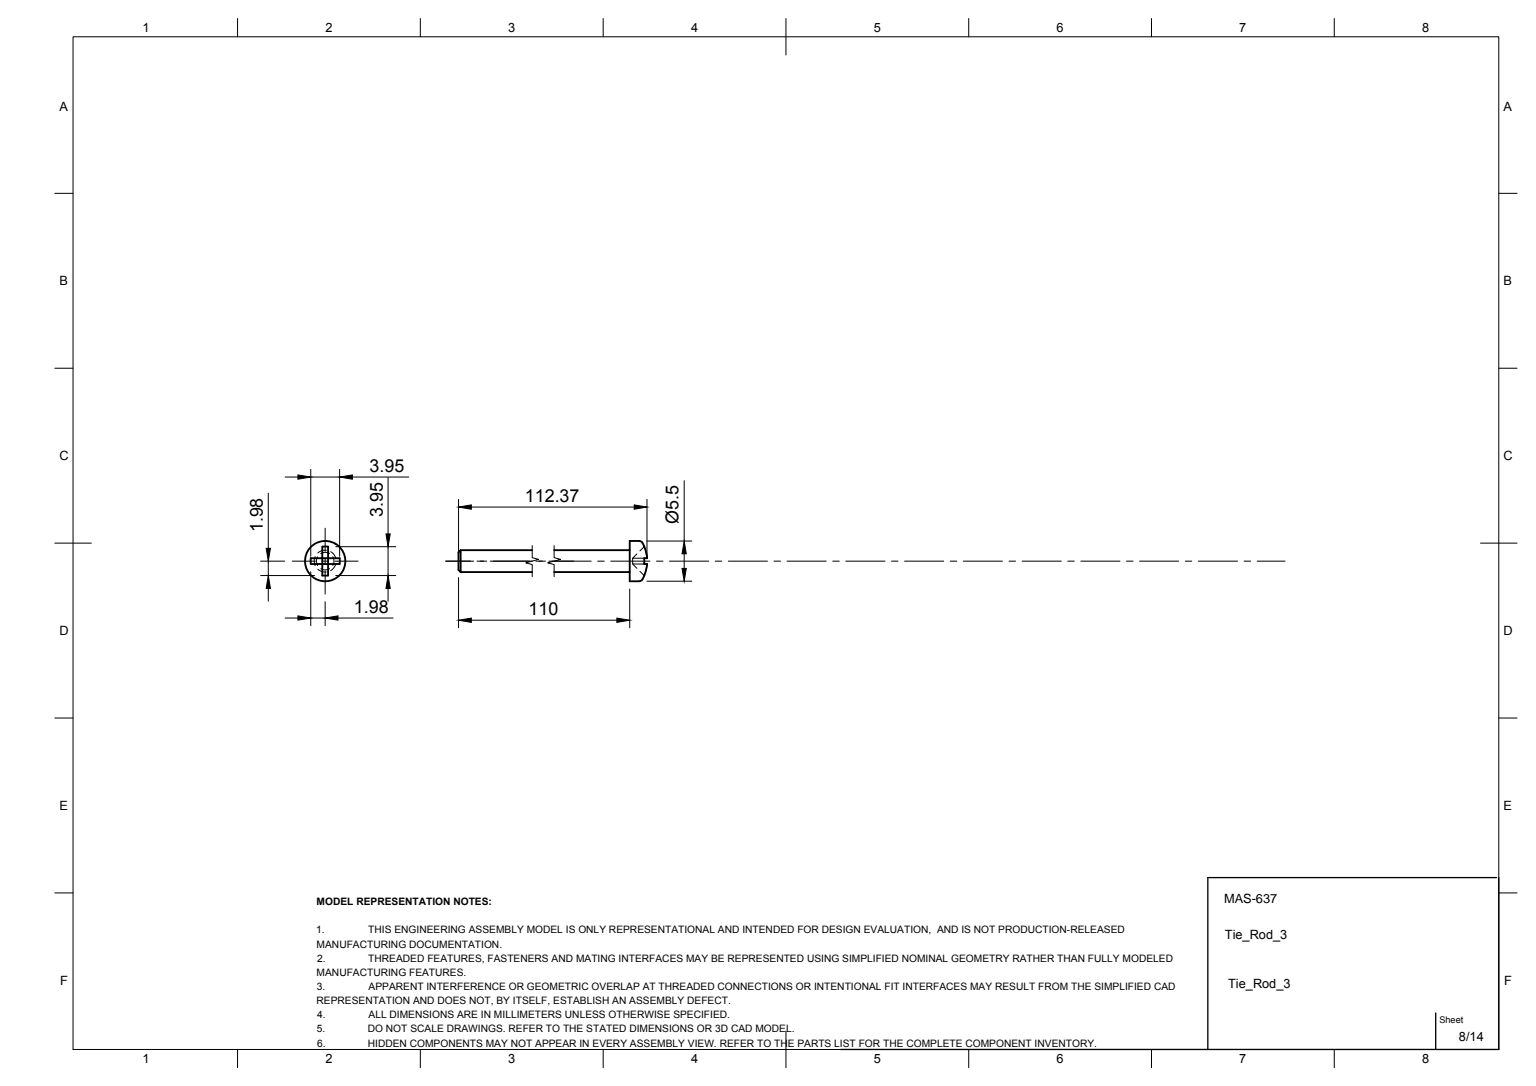
ISO-10303-21;
HEADER;
FILE_DESCRIPTION((''),'2;1');
FILE_NAME('Tie_Rod_3.step','2026-10-09T10:11:57-07:00',(''),(''),'','','');
FILE_SCHEMA (('AUTOMOTIVE_DESIGN { 1 0 10303 214 3 1 1 }'));
ENDSEC;
DATA;
#10=MECHANICAL_DESIGN_GEOMETRIC_PRESENTATION_REPRESENTATION('',(#128),#13510);
#73=SPHERICAL_SURFACE('',#8150,5.) ;
#98=SHAPE_REPRESENTATION_RELATIONSHIP('SRR','None',#13568,#113) ;
#113=ADVANCED_BREP_SHAPE_REPRESENTATION('',(#160),#13500) ;
#128=STYLED_ITEM('',(#13650),#160) ;
#160=MANIFOLD_SOLID_BREP('Body1',#7377) ;
#242=FACE_BOUND('',#1414,.T.) ;
#382=PLANE('',#8135) ;
#383=PLANE('',#8136) ;
#384=PLANE('',#8137) ;
#385=PLANE('',#8139) ;
#386=PLANE('',#8141) ;
#387=PLANE('',#8144) ;
#388=PLANE('',#8146) ;
#389=PLANE('',#8148) ;
#390=PLANE('',#8158) ;
#391=PLANE('',#8159) ;
#392=PLANE('',#8160) ;
#393=PLANE('',#8161) ;
#394=PLANE('',#8162) ;
#395=PLANE('',#8163) ;
#396=PLANE('',#8164) ;
#500=TOROIDAL_SURFACE('',#8124,2.25,0.5) ;
#636=CYLINDRICAL_SURFACE('',#8128,2.75) ;
#637=CYLINDRICAL_SURFACE('',#8130,1.5) ;
#906=FACE_OUTER_BOUND('',#1409,.T.) ;
#907=FACE_OUTER_BOUND('',#1410,.T.) ;
#908=FACE_OUTER_BOUND('',#1411,.T.) ;
#909=FACE_OUTER_BOUND('',#1412,.T.) ;
#910=FACE_OUTER_BOUND('',#1413,.T.) ;
#911=FACE_OUTER_BOUND('',#1415,.T.) ;
#912=FACE_OUTER_BOUND('',#1416,.T.) ;
#913=FACE_OUTER_BOUND('',#1417,.T.) ;
#914=FACE_OUTER_BOUND('',#1418,.T.) ;
#915=FACE_OUTER_BOUND('',#1419,.T.) ;
#916=FACE_OUTER_BOUND('',#1420,.T.) ;
#917=FACE_OUTER_BOUND('',#1421,.T.) ;
#918=FACE_OUTER_BOUND('',#1422,.T.) ;
#919=FACE_OUTER_BOUND('',#1423,.T.) ;
#920=FACE_OUTER_BOUND('',#1424,.T.) ;
#921=FACE_OUTER_BOUND('',#1425,.T.) ;
#922=FACE_OUTER_BOUND('',#1426,.T.) ;
#923=FACE_OUTER_BOUND('',#1427,.T.) ;
#924=FACE_OUTER_BOUND('',#1428,.T.) ;
#925=FACE_OUTER_BOUND('',#1429,.T.) ;
#1409=EDGE_LOOP('',(#6066,#6067,#6068,#6069)) ;
#1410=EDGE_LOOP('',(#6070,#6071,#6072,#6073)) ;
#1411=EDGE_LOOP('',(#6074,#6075,#6076,#6077)) ;
#1412=EDGE_LOOP('',(#6078,#6079,#6080,#6081)) ;
#1413=EDGE_LOOP('',(#6082)) ;
#1414=EDGE_LOOP('',(#6083)) ;
#1415=EDGE_LOOP('',(#6084)) ;
#1416=EDGE_LOOP('',(#6085,#6086,#6087,#6088)) ;
#1417=EDGE_LOOP('',(#6089,#6090,#6091,#6092)) ;
#1418=EDGE_LOOP('',(#6093,#6094,#6095,#6096)) ;
#1419=EDGE_LOOP('',(#6097,#6098,#6099)) ;
#1420=EDGE_LOOP('',(#6100,#6101,#6102)) ;
#1421=EDGE_LOOP('',(#6103,#6104,#6105)) ;
#1422=EDGE_LOOP('',(#6106,#6107,#6108,#6109,#6110,#6111,#6112,#6113,#6114,
#6115,#6116,#6117,#6118,#6119,#6120,#6121)) ;
#1423=EDGE_LOOP('',(#6122,#6123,#6124)) ;
#1424=EDGE_LOOP('',(#6125,#6126,#6127,#6128)) ;
#1425=EDGE_LOOP('',(#6129,#6130,#6131)) ;
#1426=EDGE_LOOP('',(#6132,#6133,#6134)) ;
#1427=EDGE_LOOP('',(#6135,#6136,#6137,#6138)) ;
#1428=EDGE_LOOP('',(#6139,#6140,#6141)) ;
#1429=EDGE_LOOP('',(#6142,#6143,#6144,#6145)) ;
#1944=LINE('',#12588,#2438) ;
#1945=LINE('',#12593,#2439) ;
#1946=LINE('',#12597,#2440) ;
#1947=LINE('',#12604,#2441) ;
#1948=LINE('',#12606,#2442) ;
#1949=LINE('',#12608,#2443) ;
#1950=LINE('',#12615,#2444) ;
#1951=LINE('',#12617,#2445) ;
#1952=LINE('',#12618,#2446) ;
#1953=LINE('',#12621,#2447) ;
#1954=LINE('',#12627,#2448) ;
#1955=LINE('',#12632,#2449) ;
#1956=LINE('',#12636,#2450) ;
#1957=LINE('',#12650,#2451) ;
#1958=LINE('',#12652,#2452) ;
#1959=LINE('',#12653,#2453) ;
#1960=LINE('',#12656,#2454) ;
#1961=LINE('',#12658,#2455) ;
#1962=LINE('',#12659,#2456) ;
#2438=VECTOR('',#9982,2.75) ;
#2439=VECTOR('',#9987,1.5) ;
#2440=VECTOR('',#9992,1.2) ;
#2441=VECTOR('',#10001,1.00000000000035) ;
#2442=VECTOR('',#10002,0.99999999999962) ;
#2443=VECTOR('',#10003,1.00000000000035) ;
#2444=VECTOR('',#10010,1.00000000000035) ;
#2445=VECTOR('',#10011,0.99999999999962) ;
#2446=VECTOR('',#10012,1.00000000000035) ;
#2447=VECTOR('',#10015,1.) ;
#2448=VECTOR('',#10022,1.) ;
#2449=VECTOR('',#10029,1.) ;
#2450=VECTOR('',#10034,1.) ;
#2451=VECTOR('',#10053,1.00000000000035) ;
#2452=VECTOR('',#10056,1.00000000000035) ;
#2453=VECTOR('',#10057,0.99999999999962) ;
#2454=VECTOR('',#10062,1.00000000000035) ;
#2455=VECTOR('',#10065,0.99999999999962) ;
#2456=VECTOR('',#10066,1.00000000000035) ;
#2940=CIRCLE('',#8125,2.75) ;
#2941=CIRCLE('',#8126,0.5) ;
#2942=CIRCLE('',#8127,2.5) ;
#2943=CIRCLE('',#8129,2.75) ;
#2944=CIRCLE('',#8131,1.5) ;
#2945=CIRCLE('',#8132,1.5) ;
#2946=CIRCLE('',#8134,1.2) ;
#2947=CIRCLE('',#8138,4.64997589841126) ;
#2948=CIRCLE('',#8140,4.64997589841224) ;
#2949=CIRCLE('',#8142,4.98397431775083) ;
#2950=CIRCLE('',#8143,4.98397431775083) ;
#2951=CIRCLE('',#8145,4.98396179855413) ;
#2952=CIRCLE('',#8147,4.98396179762506) ;
#2953=CIRCLE('',#8149,4.98397431775083) ;
#2954=CIRCLE('',#8151,5.) ;
#2955=CIRCLE('',#8152,4.9839743177518) ;
#2956=CIRCLE('',#8153,4.64973117502146) ;
#2957=CIRCLE('',#8154,4.98397431775041) ;
#2958=CIRCLE('',#8155,4.98397431775041) ;
#2959=CIRCLE('',#8156,4.64973117502146) ;
#2960=CIRCLE('',#8157,4.9839743177518) ;
#3542=VERTEX_POINT('',#12580) ;
#3543=VERTEX_POINT('',#12582) ;
#3544=VERTEX_POINT('',#12586) ;
#3545=VERTEX_POINT('',#12590) ;
#3546=VERTEX_POINT('',#12592) ;
#3547=VERTEX_POINT('',#12596) ;
#3548=VERTEX_POINT('',#12602) ;
#3549=VERTEX_POINT('',#12603) ;
#3550=VERTEX_POINT('',#12605) ;
#3551=VERTEX_POINT('',#12607) ;
#3552=VERTEX_POINT('',#12611) ;
#3553=VERTEX_POINT('',#12612) ;
#3554=VERTEX_POINT('',#12614) ;
#3555=VERTEX_POINT('',#12616) ;
#3556=VERTEX_POINT('',#12620) ;
#3557=VERTEX_POINT('',#12622) ;
#3558=VERTEX_POINT('',#12626) ;
#3559=VERTEX_POINT('',#12630) ;
#3560=VERTEX_POINT('',#12634) ;
#3561=VERTEX_POINT('',#12639) ;
#3562=VERTEX_POINT('',#12641) ;
#3563=VERTEX_POINT('',#12644) ;
#3564=VERTEX_POINT('',#12646) ;
#4420=EDGE_CURVE('',#3542,#3542,#2940,.T.) ;
#4421=EDGE_CURVE('',#3542,#3543,#2941,.T.) ;
#4422=EDGE_CURVE('',#3543,#3543,#2942,.T.) ;
#4423=EDGE_CURVE('',#3544,#3544,#2943,.T.) ;
#4424=EDGE_CURVE('',#3544,#3542,#1944,.T.) ;
#4425=EDGE_CURVE('',#3545,#3545,#2944,.T.) ;
#4426=EDGE_CURVE('',#3545,#3546,#1945,.T.) ;
#4427=EDGE_CURVE('',#3546,#3546,#2945,.T.) ;
#4428=EDGE_CURVE('',#3545,#3547,#1946,.T.) ;
#4429=EDGE_CURVE('',#3547,#3547,#2946,.F.) ;
#4430=EDGE_CURVE('',#3548,#3549,#1947,.T.) ;
#4431=EDGE_CURVE('',#3548,#3550,#1948,.F.) ;
#4432=EDGE_CURVE('',#3550,#3551,#1949,.T.) ;
#4433=EDGE_CURVE('',#3551,#3549,#2947,.T.) ;
#4434=EDGE_CURVE('',#3552,#3553,#2948,.T.) ;
#4435=EDGE_CURVE('',#3552,#3554,#1950,.F.) ;
#4436=EDGE_CURVE('',#3555,#3554,#1951,.F.) ;
#4437=EDGE_CURVE('',#3553,#3555,#1952,.F.) ;
#4438=EDGE_CURVE('',#3550,#3556,#1953,.T.) ;
#4439=EDGE_CURVE('',#3557,#3556,#2949,.F.) ;
#4440=EDGE_CURVE('',#3551,#3557,#2950,.F.) ;
#4441=EDGE_CURVE('',#3554,#3558,#1954,.T.) ;
#4442=EDGE_CURVE('',#3558,#3552,#2951,.T.) ;
#4443=EDGE_CURVE('',#3559,#3549,#2952,.T.) ;
#4444=EDGE_CURVE('',#3548,#3559,#1955,.T.) ;
#4445=EDGE_CURVE('',#3553,#3560,#2953,.F.) ;
#4446=EDGE_CURVE('',#3555,#3560,#1956,.T.) ;
#4447=EDGE_CURVE('',#3543,#3557,#2954,.T.) ;
#4448=EDGE_CURVE('',#3561,#3556,#2955,.T.) ;
#4449=EDGE_CURVE('',#3562,#3561,#2956,.T.) ;
#4450=EDGE_CURVE('',#3562,#3558,#2957,.T.) ;
#4451=EDGE_CURVE('',#3563,#3560,#2958,.T.) ;
#4452=EDGE_CURVE('',#3563,#3564,#2959,.T.) ;
#4453=EDGE_CURVE('',#3564,#3559,#2960,.T.) ;
#4454=EDGE_CURVE('',#3564,#3548,#1957,.F.) ;
#4455=EDGE_CURVE('',#3563,#3555,#1958,.F.) ;
#4456=EDGE_CURVE('',#3555,#3548,#1959,.T.) ;
#4457=EDGE_CURVE('',#3550,#3561,#1960,.T.) ;
#4458=EDGE_CURVE('',#3554,#3550,#1961,.T.) ;
#4459=EDGE_CURVE('',#3554,#3562,#1962,.T.) ;
#6066=ORIENTED_EDGE('',*,*,#4420,.F.) ;
#6067=ORIENTED_EDGE('',*,*,#4421,.T.) ;
#6068=ORIENTED_EDGE('',*,*,#4422,.T.) ;
#6069=ORIENTED_EDGE('',*,*,#4421,.F.) ;
#6070=ORIENTED_EDGE('',*,*,#4423,.F.) ;
#6071=ORIENTED_EDGE('',*,*,#4424,.T.) ;
#6072=ORIENTED_EDGE('',*,*,#4420,.T.) ;
#6073=ORIENTED_EDGE('',*,*,#4424,.F.) ;
#6074=ORIENTED_EDGE('',*,*,#4425,.F.) ;
#6075=ORIENTED_EDGE('',*,*,#4426,.T.) ;
#6076=ORIENTED_EDGE('',*,*,#4427,.T.) ;
#6077=ORIENTED_EDGE('',*,*,#4426,.F.) ;
#6078=ORIENTED_EDGE('',*,*,#4425,.T.) ;
#6079=ORIENTED_EDGE('',*,*,#4428,.T.) ;
#6080=ORIENTED_EDGE('',*,*,#4429,.F.) ;
#6081=ORIENTED_EDGE('',*,*,#4428,.F.) ;
#6082=ORIENTED_EDGE('',*,*,#4423,.T.) ;
#6083=ORIENTED_EDGE('',*,*,#4427,.F.) ;
#6084=ORIENTED_EDGE('',*,*,#4429,.T.) ;
#6085=ORIENTED_EDGE('',*,*,#4430,.F.) ;
#6086=ORIENTED_EDGE('',*,*,#4431,.T.) ;
#6087=ORIENTED_EDGE('',*,*,#4432,.T.) ;
#6088=ORIENTED_EDGE('',*,*,#4433,.T.) ;
#6089=ORIENTED_EDGE('',*,*,#4434,.F.) ;
#6090=ORIENTED_EDGE('',*,*,#4435,.T.) ;
#6091=ORIENTED_EDGE('',*,*,#4436,.F.) ;
#6092=ORIENTED_EDGE('',*,*,#4437,.F.) ;
#6093=ORIENTED_EDGE('',*,*,#4438,.T.) ;
#6094=ORIENTED_EDGE('',*,*,#4439,.F.) ;
#6095=ORIENTED_EDGE('',*,*,#4440,.F.) ;
#6096=ORIENTED_EDGE('',*,*,#4432,.F.) ;
#6097=ORIENTED_EDGE('',*,*,#4441,.F.) ;
#6098=ORIENTED_EDGE('',*,*,#4435,.F.) ;
#6099=ORIENTED_EDGE('',*,*,#4442,.F.) ;
#6100=ORIENTED_EDGE('',*,*,#4430,.T.) ;
#6101=ORIENTED_EDGE('',*,*,#4443,.F.) ;
#6102=ORIENTED_EDGE('',*,*,#4444,.F.) ;
#6103=ORIENTED_EDGE('',*,*,#4445,.F.) ;
#6104=ORIENTED_EDGE('',*,*,#4437,.T.) ;
#6105=ORIENTED_EDGE('',*,*,#4446,.T.) ;
#6106=ORIENTED_EDGE('',*,*,#4422,.F.) ;
#6107=ORIENTED_EDGE('',*,*,#4447,.T.) ;
#6108=ORIENTED_EDGE('',*,*,#4439,.T.) ;
#6109=ORIENTED_EDGE('',*,*,#4448,.F.) ;
#6110=ORIENTED_EDGE('',*,*,#4449,.F.) ;
#6111=ORIENTED_EDGE('',*,*,#4450,.T.) ;
#6112=ORIENTED_EDGE('',*,*,#4442,.T.) ;
#6113=ORIENTED_EDGE('',*,*,#4434,.T.) ;
#6114=ORIENTED_EDGE('',*,*,#4445,.T.) ;
#6115=ORIENTED_EDGE('',*,*,#4451,.F.) ;
#6116=ORIENTED_EDGE('',*,*,#4452,.T.) ;
#6117=ORIENTED_EDGE('',*,*,#4453,.T.) ;
#6118=ORIENTED_EDGE('',*,*,#4443,.T.) ;
#6119=ORIENTED_EDGE('',*,*,#4433,.F.) ;
#6120=ORIENTED_EDGE('',*,*,#4440,.T.) ;
#6121=ORIENTED_EDGE('',*,*,#4447,.F.) ;
#6122=ORIENTED_EDGE('',*,*,#4454,.T.) ;
#6123=ORIENTED_EDGE('',*,*,#4444,.T.) ;
#6124=ORIENTED_EDGE('',*,*,#4453,.F.) ;
#6125=ORIENTED_EDGE('',*,*,#4454,.F.) ;
#6126=ORIENTED_EDGE('',*,*,#4452,.F.) ;
#6127=ORIENTED_EDGE('',*,*,#4455,.T.) ;
#6128=ORIENTED_EDGE('',*,*,#4456,.T.) ;
#6129=ORIENTED_EDGE('',*,*,#4451,.T.) ;
#6130=ORIENTED_EDGE('',*,*,#4446,.F.) ;
#6131=ORIENTED_EDGE('',*,*,#4455,.F.) ;
#6132=ORIENTED_EDGE('',*,*,#4457,.T.) ;
#6133=ORIENTED_EDGE('',*,*,#4448,.T.) ;
#6134=ORIENTED_EDGE('',*,*,#4438,.F.) ;
#6135=ORIENTED_EDGE('',*,*,#4457,.F.) ;
#6136=ORIENTED_EDGE('',*,*,#4458,.F.) ;
#6137=ORIENTED_EDGE('',*,*,#4459,.T.) ;
#6138=ORIENTED_EDGE('',*,*,#4449,.T.) ;
#6139=ORIENTED_EDGE('',*,*,#4441,.T.) ;
#6140=ORIENTED_EDGE('',*,*,#4450,.F.) ;
#6141=ORIENTED_EDGE('',*,*,#4459,.F.) ;
#6142=ORIENTED_EDGE('',*,*,#4458,.T.) ;
#6143=ORIENTED_EDGE('',*,*,#4431,.F.) ;
#6144=ORIENTED_EDGE('',*,*,#4456,.F.) ;
#6145=ORIENTED_EDGE('',*,*,#4436,.T.) ;
#6887=CONICAL_SURFACE('',#8133,1.2,0.785398163397) ;
#7156=ADVANCED_FACE('',(#906),#500,.T.) ;
#7157=ADVANCED_FACE('',(#907),#636,.T.) ;
#7158=ADVANCED_FACE('',(#908),#637,.T.) ;
#7159=ADVANCED_FACE('',(#909),#6887,.T.) ;
#7160=ADVANCED_FACE('',(#910,#242),#382,.T.) ;
#7161=ADVANCED_FACE('',(#911),#383,.T.) ;
#7162=ADVANCED_FACE('',(#912),#384,.T.) ;
#7163=ADVANCED_FACE('',(#913),#385,.F.) ;
#7164=ADVANCED_FACE('',(#914),#386,.F.) ;
#7165=ADVANCED_FACE('',(#915),#387,.F.) ;
#7166=ADVANCED_FACE('',(#916),#388,.T.) ;
#7167=ADVANCED_FACE('',(#917),#389,.T.) ;
#7168=ADVANCED_FACE('',(#918),#73,.T.) ;
#7169=ADVANCED_FACE('',(#919),#390,.T.) ;
#7170=ADVANCED_FACE('',(#920),#391,.F.) ;
#7171=ADVANCED_FACE('',(#921),#392,.F.) ;
#7172=ADVANCED_FACE('',(#922),#393,.T.) ;
#7173=ADVANCED_FACE('',(#923),#394,.T.) ;
#7174=ADVANCED_FACE('',(#924),#395,.F.) ;
#7175=ADVANCED_FACE('',(#925),#396,.F.) ;
#7377=CLOSED_SHELL('',(#7156,#7157,#7158,#7159,#7160,#7161,#7162,#7163,
#7164,#7165,#7166,#7167,#7168,#7169,#7170,#7171,#7172,#7173,#7174,#7175)) ;
#8123=AXIS2_PLACEMENT_3D('',#12578,#9968,#9969) ;
#8124=AXIS2_PLACEMENT_3D('',#12579,#9970,#9971) ;
#8125=AXIS2_PLACEMENT_3D('',#12581,#9972,#9973) ;
#8126=AXIS2_PLACEMENT_3D('',#12583,#9974,#9975) ;
#8127=AXIS2_PLACEMENT_3D('',#12584,#9976,#9977) ;
#8128=AXIS2_PLACEMENT_3D('',#12585,#9978,#9979) ;
#8129=AXIS2_PLACEMENT_3D('',#12587,#9980,#9981) ;
#8130=AXIS2_PLACEMENT_3D('',#12589,#9983,#9984) ;
#8131=AXIS2_PLACEMENT_3D('',#12591,#9985,#9986) ;
#8132=AXIS2_PLACEMENT_3D('',#12594,#9988,#9989) ;
#8133=AXIS2_PLACEMENT_3D('',#12595,#9990,#9991) ;
#8134=AXIS2_PLACEMENT_3D('',#12598,#9993,#9994) ;
#8135=AXIS2_PLACEMENT_3D('',#12599,#9995,#9996) ;
#8136=AXIS2_PLACEMENT_3D('',#12600,#9997,#9998) ;
#8137=AXIS2_PLACEMENT_3D('',#12601,#9999,#10000) ;
#8138=AXIS2_PLACEMENT_3D('',#12609,#10004,#10005) ;
#8139=AXIS2_PLACEMENT_3D('',#12610,#10006,#10007) ;
#8140=AXIS2_PLACEMENT_3D('',#12613,#10008,#10009) ;
#8141=AXIS2_PLACEMENT_3D('',#12619,#10013,#10014) ;
#8142=AXIS2_PLACEMENT_3D('',#12623,#10016,#10017) ;
#8143=AXIS2_PLACEMENT_3D('',#12624,#10018,#10019) ;
#8144=AXIS2_PLACEMENT_3D('',#12625,#10020,#10021) ;
#8145=AXIS2_PLACEMENT_3D('',#12628,#10023,#10024) ;
#8146=AXIS2_PLACEMENT_3D('',#12629,#10025,#10026) ;
#8147=AXIS2_PLACEMENT_3D('',#12631,#10027,#10028) ;
#8148=AXIS2_PLACEMENT_3D('',#12633,#10030,#10031) ;
#8149=AXIS2_PLACEMENT_3D('',#12635,#10032,#10033) ;
#8150=AXIS2_PLACEMENT_3D('',#12637,#10035,#10036) ;
#8151=AXIS2_PLACEMENT_3D('',#12638,#10037,#10038) ;
#8152=AXIS2_PLACEMENT_3D('',#12640,#10039,#10040) ;
#8153=AXIS2_PLACEMENT_3D('',#12642,#10041,#10042) ;
#8154=AXIS2_PLACEMENT_3D('',#12643,#10043,#10044) ;
#8155=AXIS2_PLACEMENT_3D('',#12645,#10045,#10046) ;
#8156=AXIS2_PLACEMENT_3D('',#12647,#10047,#10048) ;
#8157=AXIS2_PLACEMENT_3D('',#12648,#10049,#10050) ;
#8158=AXIS2_PLACEMENT_3D('',#12649,#10051,#10052) ;
#8159=AXIS2_PLACEMENT_3D('',#12651,#10054,#10055) ;
#8160=AXIS2_PLACEMENT_3D('',#12654,#10058,#10059) ;
#8161=AXIS2_PLACEMENT_3D('',#12655,#10060,#10061) ;
#8162=AXIS2_PLACEMENT_3D('',#12657,#10063,#10064) ;
#8163=AXIS2_PLACEMENT_3D('',#12660,#10067,#10068) ;
#8164=AXIS2_PLACEMENT_3D('',#12661,#10069,#10070) ;
#9968=DIRECTION('axis',(0.,0.,1.)) ;
#9969=DIRECTION('refdir',(1.,0.,0.)) ;
#9970=DIRECTION('center_axis',(0.,0.,1.)) ;
#9971=DIRECTION('ref_axis',(0.999721561817394,-0.0235965852909097,0.)) ;
#9972=DIRECTION('center_axis',(0.,0.,1.)) ;
#9973=DIRECTION('ref_axis',(-1.,0.,0.)) ;
#9974=DIRECTION('center_axis',(-0.0235965852909095,-0.999721561817394,0.)) ;
#9975=DIRECTION('ref_axis',(-0.999721561817394,0.0235965852909095,0.)) ;
#9976=DIRECTION('center_axis',(0.,0.,1.)) ;
#9977=DIRECTION('ref_axis',(-1.,0.,0.)) ;
#9978=DIRECTION('center_axis',(0.,0.,1.)) ;
#9979=DIRECTION('ref_axis',(0.999721561817394,-0.0235965852909093,0.)) ;
#9980=DIRECTION('center_axis',(0.,0.,1.)) ;
#9981=DIRECTION('ref_axis',(-1.,0.,0.)) ;
#9982=DIRECTION('',(0.,0.,-1.)) ;
#9983=DIRECTION('center_axis',(0.,0.,1.)) ;
#9984=DIRECTION('ref_axis',(0.999721561817394,-0.0235965852909093,0.)) ;
#9985=DIRECTION('center_axis',(0.,0.,1.)) ;
#9986=DIRECTION('ref_axis',(-1.,0.,0.)) ;
#9987=DIRECTION('',(0.,0.,-1.)) ;
#9988=DIRECTION('center_axis',(0.,0.,1.)) ;
#9989=DIRECTION('ref_axis',(-1.,0.,0.)) ;
#9990=DIRECTION('center_axis',(0.,0.,-1.)) ;
#9991=DIRECTION('ref_axis',(0.999721561817394,-0.0235965852909093,0.)) ;
#9992=DIRECTION('',(0.706909895659168,-0.0166853054720413,0.707106781186865)) ;
#9993=DIRECTION('center_axis',(0.,0.,-1.)) ;
#9994=DIRECTION('ref_axis',(1.,0.,0.)) ;
#9995=DIRECTION('center_axis',(0.,0.,1.)) ;
#9996=DIRECTION('ref_axis',(1.,0.,0.)) ;
#9997=DIRECTION('center_axis',(0.,0.,1.)) ;
#9998=DIRECTION('ref_axis',(1.,0.,0.)) ;
#9999=DIRECTION('center_axis',(0.612372435695786,-0.353553390592877,-0.707106781186753)) ;
#10000=DIRECTION('ref_axis',(-0.612372435696143,0.353553390593082,-0.707106781186342)) ;
#10001=DIRECTION('',(-0.612372435695786,0.353553390592877,-0.707106781186753)) ;
#10002=DIRECTION('',(0.50000000000019,0.866025403784329,0.)) ;
#10003=DIRECTION('',(-0.612372435695786,0.353553390592877,-0.707106781186753)) ;
#10004=DIRECTION('center_axis',(0.612372436109239,-0.353553390846033,-0.707106780702115)) ;
#10005=DIRECTION('ref_axis',(-0.567091543180833,0.426740048530838,-0.704485707898095)) ;
#10006=DIRECTION('center_axis',(0.612372435695786,-0.353553390592877,0.707106781186753)) ;
#10007=DIRECTION('ref_axis',(0.612372435696143,-0.353553390593082,-0.707106781186342)) ;
#10008=DIRECTION('center_axis',(0.612372436109373,-0.35355339084611,0.70710678070196)) ;
#10009=DIRECTION('ref_axis',(0.653113494420627,-0.277745658422917,-0.70448570789825)) ;
#10010=DIRECTION('',(0.612372435695786,-0.353553390592877,-0.707106781186753)) ;
#10011=DIRECTION('',(0.50000000000019,0.866025403784329,0.)) ;
#10012=DIRECTION('',(0.612372435695786,-0.353553390592877,-0.707106781186753)) ;
#10013=DIRECTION('center_axis',(-0.50000000000019,-0.866025403784329,0.)) ;
#10014=DIRECTION('ref_axis',(0.866025403784329,-0.50000000000019,0.)) ;
#10015=DIRECTION('',(0.,0.,-1.)) ;
#10016=DIRECTION('center_axis',(0.50000000000019,0.866025403784329,0.)) ;
#10017=DIRECTION('ref_axis',(0.,0.,1.)) ;
#10018=DIRECTION('center_axis',(0.50000000000019,0.866025403784329,0.)) ;
#10019=DIRECTION('ref_axis',(0.,0.,1.)) ;
#10020=DIRECTION('center_axis',(-0.50000000000019,-0.866025403784329,0.)) ;
#10021=DIRECTION('ref_axis',(0.866025403784329,-0.50000000000019,0.)) ;
#10022=DIRECTION('',(0.,0.,-1.)) ;
#10023=DIRECTION('center_axis',(-0.499999999921223,-0.86602540382992,-3.13869580474147E-10)) ;
#10024=DIRECTION('ref_axis',(0.343296529669599,-0.198202343442237,-0.918075881270615)) ;
#10025=DIRECTION('center_axis',(-0.50000000000019,-0.866025403784329,0.)) ;
#10026=DIRECTION('ref_axis',(0.866025403784329,-0.50000000000019,0.)) ;
#10027=DIRECTION('center_axis',(0.499999999890723,0.86602540384753,-5.82829672774111E-10)) ;
#10028=DIRECTION('ref_axis',(-0.343296529827961,0.198202343232421,-0.918075881256695)) ;
#10029=DIRECTION('',(0.,0.,-1.)) ;
#10030=DIRECTION('center_axis',(-0.50000000000019,-0.866025403784329,0.)) ;
#10031=DIRECTION('ref_axis',(0.866025403784329,-0.50000000000019,0.)) ;
#10032=DIRECTION('center_axis',(-0.50000000000019,-0.866025403784329,0.)) ;
#10033=DIRECTION('ref_axis',(0.,0.,1.)) ;
#10034=DIRECTION('',(0.,0.,-1.)) ;
#10035=DIRECTION('center_axis',(0.,0.,1.)) ;
#10036=DIRECTION('ref_axis',(0.999721561817394,-0.0235965852909093,0.)) ;
#10037=DIRECTION('center_axis',(-0.023596585290909,-0.999721561817394,0.)) ;
#10038=DIRECTION('ref_axis',(-0.999721561817394,0.023596585290909,0.)) ;
#10039=DIRECTION('center_axis',(0.866025403784329,-0.50000000000019,0.)) ;
#10040=DIRECTION('ref_axis',(0.,0.,1.)) ;
#10041=DIRECTION('center_axis',(0.353553390592877,0.612372435695786,-0.707106781186753)) ;
#10042=DIRECTION('ref_axis',(1.27819621364487E-16,-0.755928946018553,-0.654653670707863)) ;
#10043=DIRECTION('center_axis',(0.866025403784329,-0.50000000000019,0.)) ;
#10044=DIRECTION('ref_axis',(0.,0.,1.)) ;
#10045=DIRECTION('center_axis',(-0.866025403784329,0.50000000000019,0.)) ;
#10046=DIRECTION('ref_axis',(0.,0.,1.)) ;
#10047=DIRECTION('center_axis',(0.353553390592877,0.612372435695786,0.707106781186753)) ;
#10048=DIRECTION('ref_axis',(-1.27819621364487E-16,0.755928946018553,-0.654653670707863)) ;
#10049=DIRECTION('center_axis',(-0.866025403784329,0.50000000000019,0.)) ;
#10050=DIRECTION('ref_axis',(0.,0.,1.)) ;
#10051=DIRECTION('center_axis',(0.866025403784329,-0.50000000000019,0.)) ;
#10052=DIRECTION('ref_axis',(0.50000000000019,0.866025403784329,0.)) ;
#10053=DIRECTION('',(0.353553390592877,0.612372435695786,-0.707106781186753)) ;
#10054=DIRECTION('center_axis',(0.353553390592877,0.612372435695786,0.707106781186753)) ;
#10055=DIRECTION('ref_axis',(0.353553390593082,0.612372435696143,-0.707106781186342)) ;
#10056=DIRECTION('',(0.353553390592877,0.612372435695786,-0.707106781186753)) ;
#10057=DIRECTION('',(-0.866025403784329,0.50000000000019,0.)) ;
#10058=DIRECTION('center_axis',(0.866025403784329,-0.50000000000019,0.)) ;
#10059=DIRECTION('ref_axis',(0.50000000000019,0.866025403784329,0.)) ;
#10060=DIRECTION('center_axis',(0.866025403784329,-0.50000000000019,0.)) ;
#10061=DIRECTION('ref_axis',(0.50000000000019,0.866025403784329,0.)) ;
#10062=DIRECTION('',(-0.353553390592877,-0.612372435695786,-0.707106781186753)) ;
#10063=DIRECTION('center_axis',(0.353553390592877,0.612372435695786,-0.707106781186753)) ;
#10064=DIRECTION('ref_axis',(-0.353553390593082,-0.612372435696143,-0.707106781186342)) ;
#10065=DIRECTION('',(-0.866025403784329,0.50000000000019,0.)) ;
#10066=DIRECTION('',(-0.353553390592877,-0.612372435695786,-0.707106781186753)) ;
#10067=DIRECTION('center_axis',(0.866025403784329,-0.50000000000019,0.)) ;
#10068=DIRECTION('ref_axis',(0.50000000000019,0.866025403784329,0.)) ;
#10069=DIRECTION('center_axis',(0.,0.,1.)) ;
#10070=DIRECTION('ref_axis',(0.,1.,0.)) ;
#12578=CARTESIAN_POINT('',(0.,0.,0.)) ;
#12579=CARTESIAN_POINT('Origin',(21.6506350946,-12.5,7.50288568297)) ;
#12580=CARTESIAN_POINT('',(18.9014007996022,-12.43510939045,7.50288568297)) ;
#12581=CARTESIAN_POINT('Origin',(21.6506350946,-12.5,7.50288568297)) ;
#12582=CARTESIAN_POINT('',(19.1513311900565,-12.4410085367727,7.06987298108)) ;
#12583=CARTESIAN_POINT('Origin',(19.4012615805109,-12.4469076830955,7.50288568297)) ;
#12584=CARTESIAN_POINT('Origin',(21.6506350946,-12.5,7.06987298108)) ;
#12585=CARTESIAN_POINT('Origin',(21.6506350946,-12.5,62.6)) ;
#12586=CARTESIAN_POINT('',(18.9014007996022,-12.43510939045,8.8)) ;
#12587=CARTESIAN_POINT('Origin',(21.6506350946,-12.5,8.8)) ;
#12588=CARTESIAN_POINT('',(18.9014007996022,-12.43510939045,62.6)) ;
#12589=CARTESIAN_POINT('Origin',(21.6506350946,-12.5,62.6)) ;
#12590=CARTESIAN_POINT('',(20.1510527518739,-12.4646051220636,118.5)) ;
#12591=CARTESIAN_POINT('Origin',(21.6506350946,-12.5,118.5)) ;
#12592=CARTESIAN_POINT('',(20.1510527518739,-12.4646051220636,8.8)) ;
#12593=CARTESIAN_POINT('',(20.1510527518739,-12.4646051220636,62.6)) ;
#12594=CARTESIAN_POINT('Origin',(21.6506350946,-12.5,8.8)) ;
#12595=CARTESIAN_POINT('Origin',(21.6506350946,-12.5,118.8)) ;
#12596=CARTESIAN_POINT('',(20.4509692204191,-12.4716840976509,118.8)) ;
#12597=CARTESIAN_POINT('',(20.4509692204191,-12.4716840976509,118.8)) ;
#12598=CARTESIAN_POINT('Origin',(21.6506350946,-12.5,118.8)) ;
#12599=CARTESIAN_POINT('Origin',(0.,26.5,8.8)) ;
#12600=CARTESIAN_POINT('Origin',(0.,25.,118.8)) ;
#12601=CARTESIAN_POINT('Origin',(21.3042249331,-12.3,8.4)) ;
#12602=CARTESIAN_POINT('',(21.5042249331,-11.9535898385,8.4)) ;
#12603=CARTESIAN_POINT('',(20.1396566358079,-11.165755954609,6.82433230687586)) ;
#12604=CARTESIAN_POINT('',(20.8219407311,-11.5596728708,7.61216606458)) ;
#12605=CARTESIAN_POINT('',(21.1042249331,-12.6464101615,8.4)) ;
#12606=CARTESIAN_POINT('',(21.4042249331,-12.1267949192,8.4)) ;
#12607=CARTESIAN_POINT('',(19.739656529,-11.8585762261,6.82433212917)) ;
#12608=CARTESIAN_POINT('',(20.4219407311,-12.2524931938,7.61216606458)) ;
#12609=CARTESIAN_POINT('Origin',(22.7766185369837,-13.1500868436552,10.1001736916713)) ;
#12610=CARTESIAN_POINT('Origin',(21.9970452561,-12.7,8.4)) ;
#12611=CARTESIAN_POINT('',(23.1616135534484,-13.834244045365,6.82433230687757)) ;
#12612=CARTESIAN_POINT('',(23.5616136602,-13.1414237739,6.82433212917)) ;
#12613=CARTESIAN_POINT('Origin',(20.5246516522163,-11.8499131563448,10.1001736916728)) ;
#12614=CARTESIAN_POINT('',(21.7970452561,-13.0464101615,8.4)) ;
#12615=CARTESIAN_POINT('',(22.4793294582,-13.4403271292,7.61216606458)) ;
#12616=CARTESIAN_POINT('',(22.1970452561,-12.3535898385,8.4)) ;
#12617=CARTESIAN_POINT('',(21.8970452561,-12.8732050808,8.4)) ;
#12618=CARTESIAN_POINT('',(22.8793294582,-12.7475068062,7.61216606458)) ;
#12619=CARTESIAN_POINT('Origin',(-0.2,-0.346410161514,0.)) ;
#12620=CARTESIAN_POINT('',(21.1042249327472,-12.6464101616267,6.43210306118471)) ;
#12621=CARTESIAN_POINT('',(21.1042249331,-12.6464101615,7.41605197605)) ;
#12622=CARTESIAN_POINT('',(20.8165355472725,-12.4803126171713,6.47010239943004)) ;
#12623=CARTESIAN_POINT('Origin',(21.4506350945998,-12.8464101615139,11.4)) ;
#12624=CARTESIAN_POINT('Origin',(21.4506350945998,-12.8464101615139,11.4)) ;
#12625=CARTESIAN_POINT('Origin',(-0.2,-0.346410161514,0.)) ;
#12626=CARTESIAN_POINT('',(21.7970452562594,-13.0464101616545,6.43210306142868)) ;
#12627=CARTESIAN_POINT('',(21.7970452561,-13.0464101615,7.41605153106)) ;
#12628=CARTESIAN_POINT('Origin',(21.4506365843505,-12.8464110235,11.3999875803367)) ;
#12629=CARTESIAN_POINT('Origin',(0.2,0.346410161514,0.)) ;
#12630=CARTESIAN_POINT('',(21.5042249329488,-11.9535898383502,6.43210306142753)) ;
#12631=CARTESIAN_POINT('Origin',(21.8506336054198,-12.1535889752702,11.3999875794143)) ;
#12632=CARTESIAN_POINT('',(21.5042249331,-11.9535898385,7.41605153106)) ;
#12633=CARTESIAN_POINT('Origin',(0.2,0.346410161514,0.)) ;
#12634=CARTESIAN_POINT('',(22.1970452564628,-12.353589838379,6.4321030611861)) ;
#12635=CARTESIAN_POINT('Origin',(21.8506350946002,-12.1535898384861,11.4)) ;
#12636=CARTESIAN_POINT('',(22.1970452561,-12.3535898385,7.41605197605)) ;
#12637=CARTESIAN_POINT('Origin',(21.6506350946,-12.5,11.4)) ;
#12638=CARTESIAN_POINT('Origin',(21.6506350946,-12.5,11.4)) ;
#12639=CARTESIAN_POINT('',(20.3163909977,-14.0109785656,6.82433212917)) ;
#12640=CARTESIAN_POINT('Origin',(21.3042249330966,-12.3000000000059,11.4)) ;
#12641=CARTESIAN_POINT('',(21.0092113210321,-14.4109785651538,6.82433212927821)) ;
#12642=CARTESIAN_POINT('Origin',(22.3006350946025,-11.3741669750747,10.0999999999932)) ;
#12643=CARTESIAN_POINT('Origin',(21.9970452561184,-12.7000000000028,11.4)) ;
#12644=CARTESIAN_POINT('',(22.9848791913391,-10.9890214349336,6.82433212927589)) ;
#12645=CARTESIAN_POINT('Origin',(21.9970452561184,-12.7000000000028,11.4)) ;
#12646=CARTESIAN_POINT('',(22.2920588685,-10.5890214344,6.82433212917)) ;
#12647=CARTESIAN_POINT('Origin',(21.0006350945975,-13.6258330249253,10.0999999999932)) ;
#12648=CARTESIAN_POINT('Origin',(21.3042249330966,-12.3000000000059,11.4)) ;
#12649=CARTESIAN_POINT('Origin',(8.8042249331,-33.9506350946,0.)) ;
#12650=CARTESIAN_POINT('',(21.8981419008,-11.2713056365,7.61216606458)) ;
#12651=CARTESIAN_POINT('Origin',(21.8506350946,-12.1535898385,8.4)) ;
#12652=CARTESIAN_POINT('',(22.5909621611,-11.6713057451,7.61216619003)) ;
#12653=CARTESIAN_POINT('',(22.0238401754,-12.2535898385,8.4)) ;
#12654=CARTESIAN_POINT('Origin',(9.49704525612,-34.3506350946,0.)) ;
#12655=CARTESIAN_POINT('Origin',(8.8042249331,-33.9506350946,0.)) ;
#12656=CARTESIAN_POINT('',(20.7103079654,-13.3286943635,7.61216606458)) ;
#12657=CARTESIAN_POINT('Origin',(21.4506350946,-12.8464101615,8.4)) ;
#12658=CARTESIAN_POINT('',(21.2774300139,-12.7464101615,8.4)) ;
#12659=CARTESIAN_POINT('',(21.4031283511,-13.7286942549,7.61216619003)) ;
#12660=CARTESIAN_POINT('Origin',(9.49704525612,-34.3506350946,0.)) ;
#12661=CARTESIAN_POINT('Origin',(0.,24.6,8.4)) ;
#13483=UNCERTAINTY_MEASURE_WITH_UNIT(LENGTH_MEASURE(0.01),#13511,
'DISTANCE_ACCURACY_VALUE',
'Maximum model space distance between geometric entities at asserted c
onnectivities') ;
#13493=UNCERTAINTY_MEASURE_WITH_UNIT(LENGTH_MEASURE(0.01),#13511,
'DISTANCE_ACCURACY_VALUE',
'Maximum model space distance between geometric entities at asserted c
onnectivities') ;
#13500=(
GEOMETRIC_REPRESENTATION_CONTEXT(3)
GLOBAL_UNCERTAINTY_ASSIGNED_CONTEXT((#13483))
GLOBAL_UNIT_ASSIGNED_CONTEXT((#13511,#13513,#13514))
REPRESENTATION_CONTEXT('','3D')
) ;
#13510=(
GEOMETRIC_REPRESENTATION_CONTEXT(3)
GLOBAL_UNCERTAINTY_ASSIGNED_CONTEXT((#13493))
GLOBAL_UNIT_ASSIGNED_CONTEXT((#13511,#13513,#13514))
REPRESENTATION_CONTEXT('','3D')
) ;
#13511=(
LENGTH_UNIT()
NAMED_UNIT(*)
SI_UNIT(.MILLI.,.METRE.)
) ;
#13513=(
NAMED_UNIT(*)
PLANE_ANGLE_UNIT()
SI_UNIT($,.RADIAN.)
) ;
#13514=(
NAMED_UNIT(*)
SI_UNIT($,.STERADIAN.)
SOLID_ANGLE_UNIT()
) ;
#13521=SHAPE_DEFINITION_REPRESENTATION(#13537,#13568) ;
#13537=PRODUCT_DEFINITION_SHAPE('',$,#13585) ;
#13568=SHAPE_REPRESENTATION('',(#8123),#13500) ;
#13578=PRODUCT_DEFINITION_CONTEXT('part definition',#13628,'design') ;
#13585=PRODUCT_DEFINITION('Tie_Rod_3','Tie_Rod_3',#13601,#13578) ;
#13601=PRODUCT_DEFINITION_FORMATION('',$,#13636) ;
#13628=APPLICATION_CONTEXT(
'Core Data for Automotive Mechanical Design Process') ;
#13629=PRODUCT_CONTEXT('part definition',#13628,'mechanical') ;
#13636=PRODUCT('Tie_Rod_3','Tie_Rod_3',$,(#13629)) ;
#13650=PRESENTATION_STYLE_ASSIGNMENT((#13655)) ;
#13655=SURFACE_STYLE_USAGE(.BOTH.,#13660) ;
#13660=SURFACE_SIDE_STYLE('',(#13665)) ;
#13665=SURFACE_STYLE_FILL_AREA(#13670) ;
#13670=FILL_AREA_STYLE('Opaque(144,144,144)',(#13675)) ;
#13675=FILL_AREA_STYLE_COLOUR('Opaque(144,144,144)',#13680) ;
#13680=COLOUR_RGB('Opaque(144,144,144)', 0.40784314, 0.44705882, 0.49803922) ;
ENDSEC;
END-ISO-10303-21;
